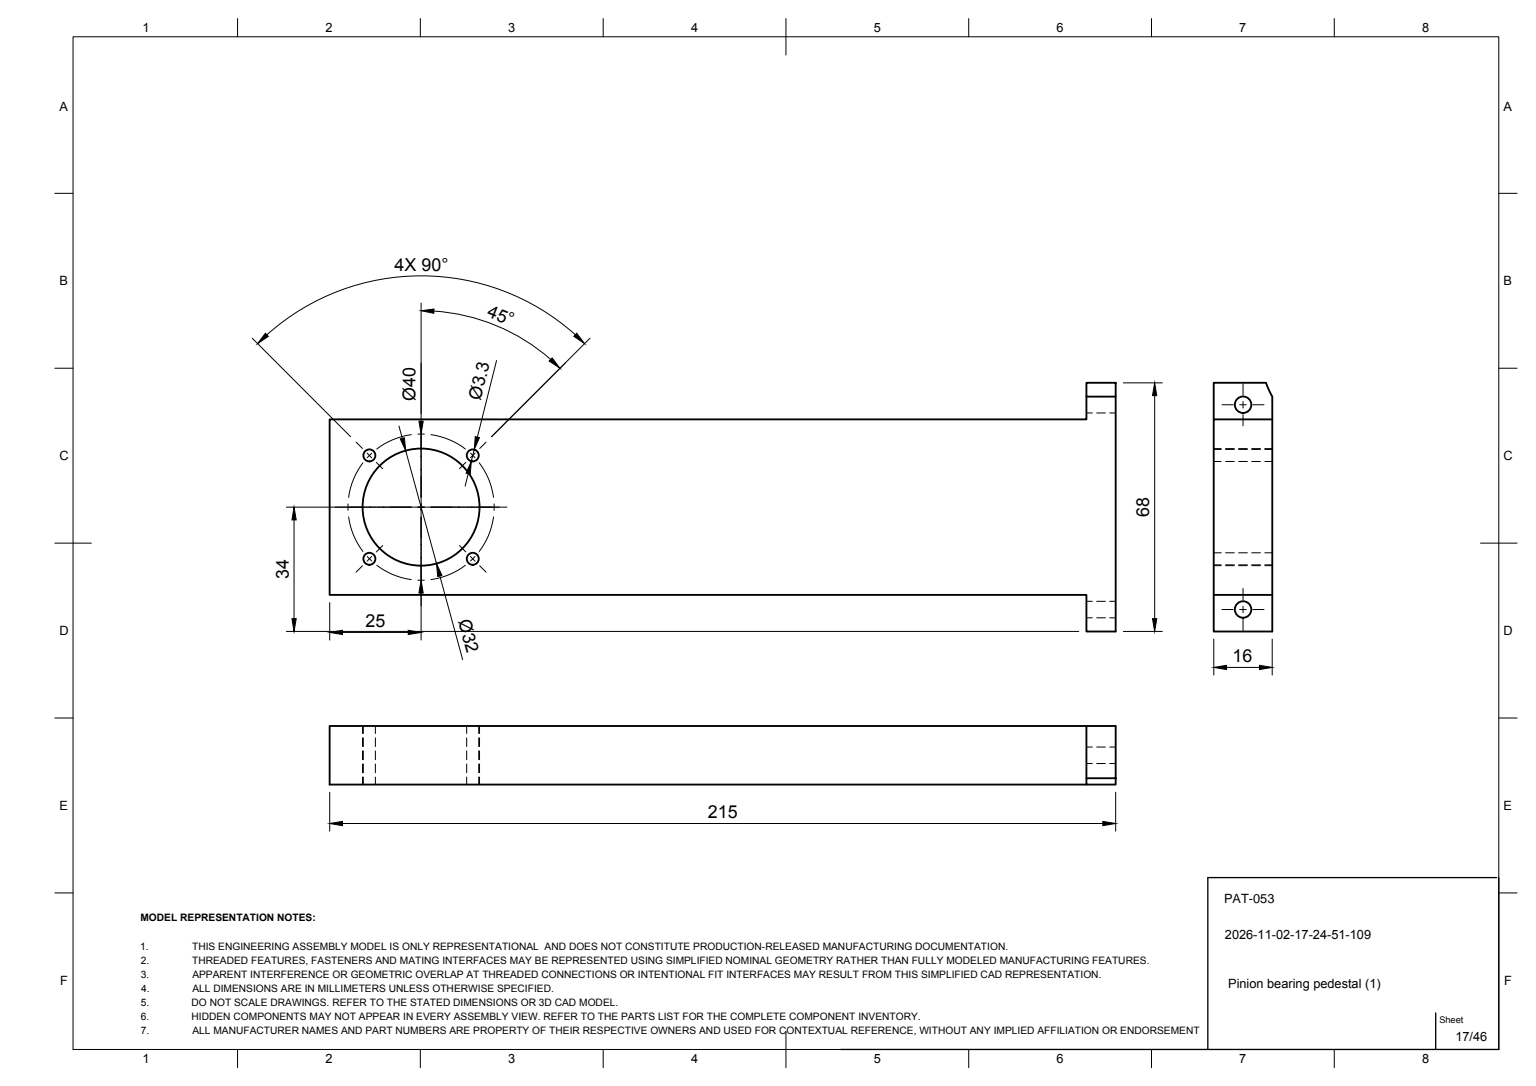
ISO-10303-21;
HEADER;
/* Generated by software containing ST-Developer
 * from STEP Tools, Inc. (www.steptools.com) 
 */

FILE_DESCRIPTION(
/* description */ ('Hand-operated arbor press'),
/* implementation_level */ '2;1');

FILE_NAME(
/* name */ 'Pinion bearing pedestal (1).step',
/* time_stamp */ '2026-10-28T03:25:25-07:00',
/* author */ (''),
/* organization */ (''),
/* preprocessor_version */ 'ST-DEVELOPER v20.2',
/* originating_system */ 'Autodesk Translation Framework v15.17.0.0',
/* authorisation */ '');

FILE_SCHEMA (('AUTOMOTIVE_DESIGN { 1 0 10303 214 3 1 1 }'));
ENDSEC;

DATA;
#10=MECHANICAL_DESIGN_GEOMETRIC_PRESENTATION_REPRESENTATION('',(#598),#32751);
#514=SHAPE_REPRESENTATION_RELATIONSHIP('SRR','None',#32943,#556);
#556=ADVANCED_BREP_SHAPE_REPRESENTATION('',(#647),#32717);
#598=STYLED_ITEM('',(#33242),#647);
#647=MANIFOLD_SOLID_BREP('Body1',#12495);
#765=FACE_BOUND('',#2225,.T.);
#766=FACE_BOUND('',#2226,.T.);
#767=FACE_BOUND('',#2228,.T.);
#768=FACE_BOUND('',#2229,.T.);
#769=FACE_BOUND('',#2230,.T.);
#770=FACE_BOUND('',#2231,.T.);
#771=FACE_BOUND('',#2232,.T.);
#772=FACE_BOUND('',#2241,.T.);
#773=FACE_BOUND('',#2243,.T.);
#774=FACE_BOUND('',#2248,.T.);
#775=FACE_BOUND('',#2249,.T.);
#776=FACE_BOUND('',#2250,.T.);
#777=FACE_BOUND('',#2251,.T.);
#778=FACE_BOUND('',#2252,.T.);
#950=PLANE('',#13307);
#951=PLANE('',#13310);
#952=PLANE('',#13330);
#953=PLANE('',#13331);
#954=PLANE('',#13332);
#955=PLANE('',#13333);
#956=PLANE('',#13334);
#957=PLANE('',#13335);
#958=PLANE('',#13336);
#959=PLANE('',#13337);
#1457=FACE_OUTER_BOUND('',#2223,.T.);
#1458=FACE_OUTER_BOUND('',#2224,.T.);
#1459=FACE_OUTER_BOUND('',#2227,.T.);
#1460=FACE_OUTER_BOUND('',#2233,.T.);
#1461=FACE_OUTER_BOUND('',#2234,.T.);
#1462=FACE_OUTER_BOUND('',#2235,.T.);
#1463=FACE_OUTER_BOUND('',#2236,.T.);
#1464=FACE_OUTER_BOUND('',#2237,.T.);
#1465=FACE_OUTER_BOUND('',#2238,.T.);
#1466=FACE_OUTER_BOUND('',#2239,.T.);
#1467=FACE_OUTER_BOUND('',#2240,.T.);
#1468=FACE_OUTER_BOUND('',#2242,.T.);
#1469=FACE_OUTER_BOUND('',#2244,.T.);
#1470=FACE_OUTER_BOUND('',#2245,.T.);
#1471=FACE_OUTER_BOUND('',#2246,.T.);
#1472=FACE_OUTER_BOUND('',#2247,.T.);
#1473=FACE_OUTER_BOUND('',#2253,.T.);
#1474=FACE_OUTER_BOUND('',#2254,.T.);
#2223=EDGE_LOOP('',(#9098,#9099,#9100,#9101));
#2224=EDGE_LOOP('',(#9102,#9103,#9104,#9105,#9106));
#2225=EDGE_LOOP('',(#9107));
#2226=EDGE_LOOP('',(#9108));
#2227=EDGE_LOOP('',(#9109,#9110,#9111,#9112,#9113,#9114,#9115,#9116));
#2228=EDGE_LOOP('',(#9117));
#2229=EDGE_LOOP('',(#9118));
#2230=EDGE_LOOP('',(#9119));
#2231=EDGE_LOOP('',(#9120));
#2232=EDGE_LOOP('',(#9121));
#2233=EDGE_LOOP('',(#9122,#9123,#9124,#9125));
#2234=EDGE_LOOP('',(#9126,#9127,#9128,#9129));
#2235=EDGE_LOOP('',(#9130,#9131,#9132,#9133));
#2236=EDGE_LOOP('',(#9134,#9135,#9136,#9137));
#2237=EDGE_LOOP('',(#9138,#9139,#9140,#9141));
#2238=EDGE_LOOP('',(#9142,#9143,#9144,#9145));
#2239=EDGE_LOOP('',(#9146,#9147,#9148,#9149));
#2240=EDGE_LOOP('',(#9150,#9151,#9152,#9153,#9154));
#2241=EDGE_LOOP('',(#9155));
#2242=EDGE_LOOP('',(#9156,#9157,#9158,#9159));
#2243=EDGE_LOOP('',(#9160));
#2244=EDGE_LOOP('',(#9161,#9162,#9163,#9164));
#2245=EDGE_LOOP('',(#9165,#9166,#9167,#9168));
#2246=EDGE_LOOP('',(#9169,#9170,#9171,#9172));
#2247=EDGE_LOOP('',(#9173,#9174,#9175,#9176,#9177,#9178,#9179,#9180));
#2248=EDGE_LOOP('',(#9181));
#2249=EDGE_LOOP('',(#9182));
#2250=EDGE_LOOP('',(#9183));
#2251=EDGE_LOOP('',(#9184));
#2252=EDGE_LOOP('',(#9185));
#2253=EDGE_LOOP('',(#9186,#9187,#9188,#9189));
#2254=EDGE_LOOP('',(#9190,#9191,#9192,#9193));
#3085=LINE('',#18467,#4256);
#3086=LINE('',#18470,#4257);
#3087=LINE('',#18473,#4258);
#3088=LINE('',#18475,#4259);
#3089=LINE('',#18477,#4260);
#3090=LINE('',#18478,#4261);
#3091=LINE('',#18485,#4262);
#3092=LINE('',#18487,#4263);
#3093=LINE('',#18489,#4264);
#3094=LINE('',#18491,#4265);
#3095=LINE('',#18493,#4266);
#3096=LINE('',#18494,#4267);
#3097=LINE('',#18507,#4268);
#3098=LINE('',#18511,#4269);
#3099=LINE('',#18515,#4270);
#3100=LINE('',#18519,#4271);
#3101=LINE('',#18523,#4272);
#3102=LINE('',#18527,#4273);
#3103=LINE('',#18531,#4274);
#3104=LINE('',#18535,#4275);
#3105=LINE('',#18537,#4276);
#3106=LINE('',#18538,#4277);
#3107=LINE('',#18541,#4278);
#3108=LINE('',#18543,#4279);
#3109=LINE('',#18544,#4280);
#3110=LINE('',#18546,#4281);
#3111=LINE('',#18548,#4282);
#3112=LINE('',#18551,#4283);
#3113=LINE('',#18552,#4284);
#3114=LINE('',#18555,#4285);
#3115=LINE('',#18556,#4286);
#3116=LINE('',#18558,#4287);
#4256=VECTOR('',#15030,1.);
#4257=VECTOR('',#15033,1.);
#4258=VECTOR('',#15036,1.);
#4259=VECTOR('',#15037,1.);
#4260=VECTOR('',#15038,1.);
#4261=VECTOR('',#15039,1.);
#4262=VECTOR('',#15046,1.);
#4263=VECTOR('',#15047,1.);
#4264=VECTOR('',#15048,1.);
#4265=VECTOR('',#15049,1.);
#4266=VECTOR('',#15050,1.);
#4267=VECTOR('',#15051,1.);
#4268=VECTOR('',#15064,0.165);
#4269=VECTOR('',#15069,0.165);
#4270=VECTOR('',#15074,0.165);
#4271=VECTOR('',#15079,0.165);
#4272=VECTOR('',#15084,0.225);
#4273=VECTOR('',#15089,0.225);
#4274=VECTOR('',#15094,1.6);
#4275=VECTOR('',#15099,1.);
#4276=VECTOR('',#15100,1.);
#4277=VECTOR('',#15101,1.);
#4278=VECTOR('',#15104,1.);
#4279=VECTOR('',#15105,1.);
#4280=VECTOR('',#15106,1.);
#4281=VECTOR('',#15109,1.);
#4282=VECTOR('',#15112,1.);
#4283=VECTOR('',#15115,1.);
#4284=VECTOR('',#15116,1.);
#4285=VECTOR('',#15119,1.);
#4286=VECTOR('',#15120,1.);
#4287=VECTOR('',#15123,1.);
#5292=CIRCLE('',#13305,2.52);
#5293=CIRCLE('',#13306,2.52);
#5294=CIRCLE('',#13308,0.225);
#5295=CIRCLE('',#13309,0.225);
#5296=CIRCLE('',#13311,0.165);
#5297=CIRCLE('',#13312,0.165);
#5298=CIRCLE('',#13313,0.165);
#5299=CIRCLE('',#13314,0.165);
#5300=CIRCLE('',#13315,1.6);
#5301=CIRCLE('',#13317,0.165);
#5302=CIRCLE('',#13319,0.165);
#5303=CIRCLE('',#13321,0.165);
#5304=CIRCLE('',#13323,0.165);
#5305=CIRCLE('',#13325,0.225);
#5306=CIRCLE('',#13327,0.225);
#5307=CIRCLE('',#13329,1.6);
#5814=VERTEX_POINT('',#18463);
#5815=VERTEX_POINT('',#18464);
#5816=VERTEX_POINT('',#18466);
#5817=VERTEX_POINT('',#18468);
#5818=VERTEX_POINT('',#18472);
#5819=VERTEX_POINT('',#18474);
#5820=VERTEX_POINT('',#18476);
#5821=VERTEX_POINT('',#18479);
#5822=VERTEX_POINT('',#18481);
#5823=VERTEX_POINT('',#18484);
#5824=VERTEX_POINT('',#18486);
#5825=VERTEX_POINT('',#18488);
#5826=VERTEX_POINT('',#18490);
#5827=VERTEX_POINT('',#18492);
#5828=VERTEX_POINT('',#18495);
#5829=VERTEX_POINT('',#18497);
#5830=VERTEX_POINT('',#18499);
#5831=VERTEX_POINT('',#18501);
#5832=VERTEX_POINT('',#18503);
#5833=VERTEX_POINT('',#18506);
#5834=VERTEX_POINT('',#18510);
#5835=VERTEX_POINT('',#18514);
#5836=VERTEX_POINT('',#18518);
#5837=VERTEX_POINT('',#18522);
#5838=VERTEX_POINT('',#18526);
#5839=VERTEX_POINT('',#18530);
#5840=VERTEX_POINT('',#18534);
#5841=VERTEX_POINT('',#18536);
#5842=VERTEX_POINT('',#18540);
#5843=VERTEX_POINT('',#18542);
#5844=VERTEX_POINT('',#18550);
#5845=VERTEX_POINT('',#18554);
#7052=EDGE_CURVE('',#5814,#5815,#5292,.T.);
#7053=EDGE_CURVE('',#5816,#5814,#3085,.T.);
#7054=EDGE_CURVE('',#5817,#5816,#5293,.T.);
#7055=EDGE_CURVE('',#5815,#5817,#3086,.T.);
#7056=EDGE_CURVE('',#5818,#5816,#3087,.T.);
#7057=EDGE_CURVE('',#5818,#5819,#3088,.T.);
#7058=EDGE_CURVE('',#5820,#5819,#3089,.T.);
#7059=EDGE_CURVE('',#5817,#5820,#3090,.T.);
#7060=EDGE_CURVE('',#5821,#5821,#5294,.T.);
#7061=EDGE_CURVE('',#5822,#5822,#5295,.T.);
#7062=EDGE_CURVE('',#5814,#5823,#3091,.T.);
#7063=EDGE_CURVE('',#5823,#5824,#3092,.T.);
#7064=EDGE_CURVE('',#5825,#5824,#3093,.T.);
#7065=EDGE_CURVE('',#5826,#5825,#3094,.T.);
#7066=EDGE_CURVE('',#5826,#5827,#3095,.T.);
#7067=EDGE_CURVE('',#5827,#5818,#3096,.T.);
#7068=EDGE_CURVE('',#5828,#5828,#5296,.T.);
#7069=EDGE_CURVE('',#5829,#5829,#5297,.T.);
#7070=EDGE_CURVE('',#5830,#5830,#5298,.T.);
#7071=EDGE_CURVE('',#5831,#5831,#5299,.T.);
#7072=EDGE_CURVE('',#5832,#5832,#5300,.T.);
#7073=EDGE_CURVE('',#5828,#5833,#3097,.T.);
#7074=EDGE_CURVE('',#5833,#5833,#5301,.T.);
#7075=EDGE_CURVE('',#5829,#5834,#3098,.T.);
#7076=EDGE_CURVE('',#5834,#5834,#5302,.T.);
#7077=EDGE_CURVE('',#5830,#5835,#3099,.T.);
#7078=EDGE_CURVE('',#5835,#5835,#5303,.T.);
#7079=EDGE_CURVE('',#5831,#5836,#3100,.T.);
#7080=EDGE_CURVE('',#5836,#5836,#5304,.T.);
#7081=EDGE_CURVE('',#5822,#5837,#3101,.T.);
#7082=EDGE_CURVE('',#5837,#5837,#5305,.T.);
#7083=EDGE_CURVE('',#5821,#5838,#3102,.T.);
#7084=EDGE_CURVE('',#5838,#5838,#5306,.T.);
#7085=EDGE_CURVE('',#5832,#5839,#3103,.T.);
#7086=EDGE_CURVE('',#5839,#5839,#5307,.T.);
#7087=EDGE_CURVE('',#5815,#5840,#3104,.T.);
#7088=EDGE_CURVE('',#5841,#5840,#3105,.T.);
#7089=EDGE_CURVE('',#5823,#5841,#3106,.T.);
#7090=EDGE_CURVE('',#5842,#5826,#3107,.T.);
#7091=EDGE_CURVE('',#5843,#5842,#3108,.T.);
#7092=EDGE_CURVE('',#5827,#5843,#3109,.T.);
#7093=EDGE_CURVE('',#5819,#5843,#3110,.T.);
#7094=EDGE_CURVE('',#5840,#5820,#3111,.T.);
#7095=EDGE_CURVE('',#5841,#5844,#3112,.T.);
#7096=EDGE_CURVE('',#5824,#5844,#3113,.T.);
#7097=EDGE_CURVE('',#5842,#5845,#3114,.T.);
#7098=EDGE_CURVE('',#5844,#5845,#3115,.T.);
#7099=EDGE_CURVE('',#5845,#5825,#3116,.T.);
#9098=ORIENTED_EDGE('',*,*,#7052,.F.);
#9099=ORIENTED_EDGE('',*,*,#7053,.F.);
#9100=ORIENTED_EDGE('',*,*,#7054,.F.);
#9101=ORIENTED_EDGE('',*,*,#7055,.F.);
#9102=ORIENTED_EDGE('',*,*,#7054,.T.);
#9103=ORIENTED_EDGE('',*,*,#7056,.F.);
#9104=ORIENTED_EDGE('',*,*,#7057,.T.);
#9105=ORIENTED_EDGE('',*,*,#7058,.F.);
#9106=ORIENTED_EDGE('',*,*,#7059,.F.);
#9107=ORIENTED_EDGE('',*,*,#7060,.T.);
#9108=ORIENTED_EDGE('',*,*,#7061,.T.);
#9109=ORIENTED_EDGE('',*,*,#7053,.T.);
#9110=ORIENTED_EDGE('',*,*,#7062,.T.);
#9111=ORIENTED_EDGE('',*,*,#7063,.T.);
#9112=ORIENTED_EDGE('',*,*,#7064,.F.);
#9113=ORIENTED_EDGE('',*,*,#7065,.F.);
#9114=ORIENTED_EDGE('',*,*,#7066,.T.);
#9115=ORIENTED_EDGE('',*,*,#7067,.T.);
#9116=ORIENTED_EDGE('',*,*,#7056,.T.);
#9117=ORIENTED_EDGE('',*,*,#7068,.T.);
#9118=ORIENTED_EDGE('',*,*,#7069,.T.);
#9119=ORIENTED_EDGE('',*,*,#7070,.T.);
#9120=ORIENTED_EDGE('',*,*,#7071,.T.);
#9121=ORIENTED_EDGE('',*,*,#7072,.T.);
#9122=ORIENTED_EDGE('',*,*,#7068,.F.);
#9123=ORIENTED_EDGE('',*,*,#7073,.T.);
#9124=ORIENTED_EDGE('',*,*,#7074,.F.);
#9125=ORIENTED_EDGE('',*,*,#7073,.F.);
#9126=ORIENTED_EDGE('',*,*,#7069,.F.);
#9127=ORIENTED_EDGE('',*,*,#7075,.T.);
#9128=ORIENTED_EDGE('',*,*,#7076,.F.);
#9129=ORIENTED_EDGE('',*,*,#7075,.F.);
#9130=ORIENTED_EDGE('',*,*,#7070,.F.);
#9131=ORIENTED_EDGE('',*,*,#7077,.T.);
#9132=ORIENTED_EDGE('',*,*,#7078,.F.);
#9133=ORIENTED_EDGE('',*,*,#7077,.F.);
#9134=ORIENTED_EDGE('',*,*,#7071,.F.);
#9135=ORIENTED_EDGE('',*,*,#7079,.T.);
#9136=ORIENTED_EDGE('',*,*,#7080,.F.);
#9137=ORIENTED_EDGE('',*,*,#7079,.F.);
#9138=ORIENTED_EDGE('',*,*,#7061,.F.);
#9139=ORIENTED_EDGE('',*,*,#7081,.T.);
#9140=ORIENTED_EDGE('',*,*,#7082,.F.);
#9141=ORIENTED_EDGE('',*,*,#7081,.F.);
#9142=ORIENTED_EDGE('',*,*,#7060,.F.);
#9143=ORIENTED_EDGE('',*,*,#7083,.T.);
#9144=ORIENTED_EDGE('',*,*,#7084,.F.);
#9145=ORIENTED_EDGE('',*,*,#7083,.F.);
#9146=ORIENTED_EDGE('',*,*,#7072,.F.);
#9147=ORIENTED_EDGE('',*,*,#7085,.T.);
#9148=ORIENTED_EDGE('',*,*,#7086,.F.);
#9149=ORIENTED_EDGE('',*,*,#7085,.F.);
#9150=ORIENTED_EDGE('',*,*,#7052,.T.);
#9151=ORIENTED_EDGE('',*,*,#7087,.T.);
#9152=ORIENTED_EDGE('',*,*,#7088,.F.);
#9153=ORIENTED_EDGE('',*,*,#7089,.F.);
#9154=ORIENTED_EDGE('',*,*,#7062,.F.);
#9155=ORIENTED_EDGE('',*,*,#7084,.T.);
#9156=ORIENTED_EDGE('',*,*,#7090,.F.);
#9157=ORIENTED_EDGE('',*,*,#7091,.F.);
#9158=ORIENTED_EDGE('',*,*,#7092,.F.);
#9159=ORIENTED_EDGE('',*,*,#7066,.F.);
#9160=ORIENTED_EDGE('',*,*,#7082,.T.);
#9161=ORIENTED_EDGE('',*,*,#7067,.F.);
#9162=ORIENTED_EDGE('',*,*,#7092,.T.);
#9163=ORIENTED_EDGE('',*,*,#7093,.F.);
#9164=ORIENTED_EDGE('',*,*,#7057,.F.);
#9165=ORIENTED_EDGE('',*,*,#7055,.T.);
#9166=ORIENTED_EDGE('',*,*,#7059,.T.);
#9167=ORIENTED_EDGE('',*,*,#7094,.F.);
#9168=ORIENTED_EDGE('',*,*,#7087,.F.);
#9169=ORIENTED_EDGE('',*,*,#7089,.T.);
#9170=ORIENTED_EDGE('',*,*,#7095,.T.);
#9171=ORIENTED_EDGE('',*,*,#7096,.F.);
#9172=ORIENTED_EDGE('',*,*,#7063,.F.);
#9173=ORIENTED_EDGE('',*,*,#7097,.T.);
#9174=ORIENTED_EDGE('',*,*,#7098,.F.);
#9175=ORIENTED_EDGE('',*,*,#7095,.F.);
#9176=ORIENTED_EDGE('',*,*,#7088,.T.);
#9177=ORIENTED_EDGE('',*,*,#7094,.T.);
#9178=ORIENTED_EDGE('',*,*,#7058,.T.);
#9179=ORIENTED_EDGE('',*,*,#7093,.T.);
#9180=ORIENTED_EDGE('',*,*,#7091,.T.);
#9181=ORIENTED_EDGE('',*,*,#7086,.T.);
#9182=ORIENTED_EDGE('',*,*,#7080,.T.);
#9183=ORIENTED_EDGE('',*,*,#7078,.T.);
#9184=ORIENTED_EDGE('',*,*,#7076,.T.);
#9185=ORIENTED_EDGE('',*,*,#7074,.T.);
#9186=ORIENTED_EDGE('',*,*,#7090,.T.);
#9187=ORIENTED_EDGE('',*,*,#7065,.T.);
#9188=ORIENTED_EDGE('',*,*,#7099,.F.);
#9189=ORIENTED_EDGE('',*,*,#7097,.F.);
#9190=ORIENTED_EDGE('',*,*,#7099,.T.);
#9191=ORIENTED_EDGE('',*,*,#7064,.T.);
#9192=ORIENTED_EDGE('',*,*,#7096,.T.);
#9193=ORIENTED_EDGE('',*,*,#7098,.T.);
#11705=CYLINDRICAL_SURFACE('',#13304,2.52);
#11706=CYLINDRICAL_SURFACE('',#13316,0.165);
#11707=CYLINDRICAL_SURFACE('',#13318,0.165);
#11708=CYLINDRICAL_SURFACE('',#13320,0.165);
#11709=CYLINDRICAL_SURFACE('',#13322,0.165);
#11710=CYLINDRICAL_SURFACE('',#13324,0.225);
#11711=CYLINDRICAL_SURFACE('',#13326,0.225);
#11712=CYLINDRICAL_SURFACE('',#13328,1.6);
#11966=ADVANCED_FACE('',(#1457),#11705,.F.);
#11967=ADVANCED_FACE('',(#1458,#765,#766),#950,.F.);
#11968=ADVANCED_FACE('',(#1459,#767,#768,#769,#770,#771),#951,.T.);
#11969=ADVANCED_FACE('',(#1460),#11706,.F.);
#11970=ADVANCED_FACE('',(#1461),#11707,.F.);
#11971=ADVANCED_FACE('',(#1462),#11708,.F.);
#11972=ADVANCED_FACE('',(#1463),#11709,.F.);
#11973=ADVANCED_FACE('',(#1464),#11710,.F.);
#11974=ADVANCED_FACE('',(#1465),#11711,.F.);
#11975=ADVANCED_FACE('',(#1466),#11712,.F.);
#11976=ADVANCED_FACE('',(#1467,#772),#952,.T.);
#11977=ADVANCED_FACE('',(#1468,#773),#953,.T.);
#11978=ADVANCED_FACE('',(#1469),#954,.T.);
#11979=ADVANCED_FACE('',(#1470),#955,.T.);
#11980=ADVANCED_FACE('',(#1471),#956,.T.);
#11981=ADVANCED_FACE('',(#1472,#774,#775,#776,#777,#778),#957,.T.);
#11982=ADVANCED_FACE('',(#1473),#958,.T.);
#11983=ADVANCED_FACE('',(#1474),#959,.T.);
#12495=CLOSED_SHELL('',(#11966,#11967,#11968,#11969,#11970,#11971,#11972,
#11973,#11974,#11975,#11976,#11977,#11978,#11979,#11980,#11981,#11982,#11983));
#13303=AXIS2_PLACEMENT_3D('',#18461,#15024,#15025);
#13304=AXIS2_PLACEMENT_3D('',#18462,#15026,#15027);
#13305=AXIS2_PLACEMENT_3D('',#18465,#15028,#15029);
#13306=AXIS2_PLACEMENT_3D('',#18469,#15031,#15032);
#13307=AXIS2_PLACEMENT_3D('',#18471,#15034,#15035);
#13308=AXIS2_PLACEMENT_3D('',#18480,#15040,#15041);
#13309=AXIS2_PLACEMENT_3D('',#18482,#15042,#15043);
#13310=AXIS2_PLACEMENT_3D('',#18483,#15044,#15045);
#13311=AXIS2_PLACEMENT_3D('',#18496,#15052,#15053);
#13312=AXIS2_PLACEMENT_3D('',#18498,#15054,#15055);
#13313=AXIS2_PLACEMENT_3D('',#18500,#15056,#15057);
#13314=AXIS2_PLACEMENT_3D('',#18502,#15058,#15059);
#13315=AXIS2_PLACEMENT_3D('',#18504,#15060,#15061);
#13316=AXIS2_PLACEMENT_3D('',#18505,#15062,#15063);
#13317=AXIS2_PLACEMENT_3D('',#18508,#15065,#15066);
#13318=AXIS2_PLACEMENT_3D('',#18509,#15067,#15068);
#13319=AXIS2_PLACEMENT_3D('',#18512,#15070,#15071);
#13320=AXIS2_PLACEMENT_3D('',#18513,#15072,#15073);
#13321=AXIS2_PLACEMENT_3D('',#18516,#15075,#15076);
#13322=AXIS2_PLACEMENT_3D('',#18517,#15077,#15078);
#13323=AXIS2_PLACEMENT_3D('',#18520,#15080,#15081);
#13324=AXIS2_PLACEMENT_3D('',#18521,#15082,#15083);
#13325=AXIS2_PLACEMENT_3D('',#18524,#15085,#15086);
#13326=AXIS2_PLACEMENT_3D('',#18525,#15087,#15088);
#13327=AXIS2_PLACEMENT_3D('',#18528,#15090,#15091);
#13328=AXIS2_PLACEMENT_3D('',#18529,#15092,#15093);
#13329=AXIS2_PLACEMENT_3D('',#18532,#15095,#15096);
#13330=AXIS2_PLACEMENT_3D('',#18533,#15097,#15098);
#13331=AXIS2_PLACEMENT_3D('',#18539,#15102,#15103);
#13332=AXIS2_PLACEMENT_3D('',#18545,#15107,#15108);
#13333=AXIS2_PLACEMENT_3D('',#18547,#15110,#15111);
#13334=AXIS2_PLACEMENT_3D('',#18549,#15113,#15114);
#13335=AXIS2_PLACEMENT_3D('',#18553,#15117,#15118);
#13336=AXIS2_PLACEMENT_3D('',#18557,#15121,#15122);
#13337=AXIS2_PLACEMENT_3D('',#18559,#15124,#15125);
#15024=DIRECTION('axis',(0.,0.,1.));
#15025=DIRECTION('refdir',(1.,0.,0.));
#15026=DIRECTION('center_axis',(0.,0.,1.));
#15027=DIRECTION('ref_axis',(1.,0.,0.));
#15028=DIRECTION('center_axis',(0.,0.,-1.));
#15029=DIRECTION('ref_axis',(1.,0.,0.));
#15030=DIRECTION('',(0.,0.,1.));
#15031=DIRECTION('center_axis',(0.,0.,1.));
#15032=DIRECTION('ref_axis',(1.,0.,0.));
#15033=DIRECTION('',(0.,0.,-1.));
#15034=DIRECTION('center_axis',(0.,0.,1.));
#15035=DIRECTION('ref_axis',(1.,0.,0.));
#15036=DIRECTION('',(1.,0.,0.));
#15037=DIRECTION('',(0.,1.,0.));
#15038=DIRECTION('',(-1.,0.,0.));
#15039=DIRECTION('',(0.,1.,0.));
#15040=DIRECTION('center_axis',(0.,0.,1.));
#15041=DIRECTION('ref_axis',(1.,0.,0.));
#15042=DIRECTION('center_axis',(0.,0.,1.));
#15043=DIRECTION('ref_axis',(1.,0.,0.));
#15044=DIRECTION('center_axis',(0.,-1.,0.));
#15045=DIRECTION('ref_axis',(1.,0.,0.));
#15046=DIRECTION('',(-1.,0.,0.));
#15047=DIRECTION('',(0.,0.,1.));
#15048=DIRECTION('',(1.,0.,0.));
#15049=DIRECTION('',(0.,0.,1.));
#15050=DIRECTION('',(-1.,0.,0.));
#15051=DIRECTION('',(0.,0.,-1.));
#15052=DIRECTION('center_axis',(0.,1.,0.));
#15053=DIRECTION('ref_axis',(1.,0.,0.));
#15054=DIRECTION('center_axis',(0.,1.,0.));
#15055=DIRECTION('ref_axis',(1.,0.,0.));
#15056=DIRECTION('center_axis',(0.,1.,0.));
#15057=DIRECTION('ref_axis',(1.,0.,0.));
#15058=DIRECTION('center_axis',(0.,1.,0.));
#15059=DIRECTION('ref_axis',(1.,0.,0.));
#15060=DIRECTION('center_axis',(0.,1.,0.));
#15061=DIRECTION('ref_axis',(1.,0.,0.));
#15062=DIRECTION('center_axis',(0.,1.,0.));
#15063=DIRECTION('ref_axis',(1.,0.,0.));
#15064=DIRECTION('',(0.,1.,0.));
#15065=DIRECTION('center_axis',(0.,-1.,0.));
#15066=DIRECTION('ref_axis',(1.,0.,0.));
#15067=DIRECTION('center_axis',(0.,1.,0.));
#15068=DIRECTION('ref_axis',(1.,0.,0.));
#15069=DIRECTION('',(0.,1.,0.));
#15070=DIRECTION('center_axis',(0.,-1.,0.));
#15071=DIRECTION('ref_axis',(1.,0.,0.));
#15072=DIRECTION('center_axis',(0.,1.,0.));
#15073=DIRECTION('ref_axis',(1.,0.,0.));
#15074=DIRECTION('',(0.,1.,0.));
#15075=DIRECTION('center_axis',(0.,-1.,0.));
#15076=DIRECTION('ref_axis',(1.,0.,0.));
#15077=DIRECTION('center_axis',(0.,1.,0.));
#15078=DIRECTION('ref_axis',(1.,0.,0.));
#15079=DIRECTION('',(0.,1.,0.));
#15080=DIRECTION('center_axis',(0.,-1.,0.));
#15081=DIRECTION('ref_axis',(1.,0.,0.));
#15082=DIRECTION('center_axis',(0.,0.,1.));
#15083=DIRECTION('ref_axis',(1.,0.,0.));
#15084=DIRECTION('',(0.,0.,1.));
#15085=DIRECTION('center_axis',(0.,0.,-1.));
#15086=DIRECTION('ref_axis',(1.,0.,0.));
#15087=DIRECTION('center_axis',(0.,0.,1.));
#15088=DIRECTION('ref_axis',(1.,0.,0.));
#15089=DIRECTION('',(0.,0.,1.));
#15090=DIRECTION('center_axis',(0.,0.,-1.));
#15091=DIRECTION('ref_axis',(1.,0.,0.));
#15092=DIRECTION('center_axis',(0.,1.,0.));
#15093=DIRECTION('ref_axis',(1.,0.,0.));
#15094=DIRECTION('',(0.,1.,0.));
#15095=DIRECTION('center_axis',(0.,-1.,0.));
#15096=DIRECTION('ref_axis',(1.,0.,0.));
#15097=DIRECTION('center_axis',(0.,0.,1.));
#15098=DIRECTION('ref_axis',(1.,0.,0.));
#15099=DIRECTION('',(0.,1.,0.));
#15100=DIRECTION('',(1.,0.,0.));
#15101=DIRECTION('',(0.,1.,0.));
#15102=DIRECTION('center_axis',(0.,0.,1.));
#15103=DIRECTION('ref_axis',(1.,0.,0.));
#15104=DIRECTION('',(0.,-1.,0.));
#15105=DIRECTION('',(1.,0.,0.));
#15106=DIRECTION('',(0.,1.,0.));
#15107=DIRECTION('center_axis',(-1.,0.,0.));
#15108=DIRECTION('ref_axis',(0.,0.,1.));
#15109=DIRECTION('',(0.,0.,1.));
#15110=DIRECTION('center_axis',(1.,0.,0.));
#15111=DIRECTION('ref_axis',(0.,0.,-1.));
#15112=DIRECTION('',(0.,0.,-1.));
#15113=DIRECTION('center_axis',(1.,0.,0.));
#15114=DIRECTION('ref_axis',(0.,1.,0.));
#15115=DIRECTION('',(0.,0.,1.));
#15116=DIRECTION('',(0.,1.,0.));
#15117=DIRECTION('center_axis',(0.,1.,0.));
#15118=DIRECTION('ref_axis',(-1.,0.,0.));
#15119=DIRECTION('',(0.,0.,1.));
#15120=DIRECTION('',(-1.,0.,0.));
#15121=DIRECTION('center_axis',(-1.,0.,0.));
#15122=DIRECTION('ref_axis',(0.,-1.,0.));
#15123=DIRECTION('',(0.,-1.,0.));
#15124=DIRECTION('center_axis',(0.,0.,1.));
#15125=DIRECTION('ref_axis',(1.,0.,0.));
#18461=CARTESIAN_POINT('',(0.,0.,0.));
#18462=CARTESIAN_POINT('Origin',(1.,0.,0.9));
#18463=CARTESIAN_POINT('',(-0.228983319658977,2.2,1.8));
#18464=CARTESIAN_POINT('',(0.15,2.37231954002828,1.8));
#18465=CARTESIAN_POINT('Origin',(1.,0.,1.8));
#18466=CARTESIAN_POINT('',(-0.228983319658977,2.2,1.));
#18467=CARTESIAN_POINT('',(-0.228983319658977,2.2,0.9));
#18468=CARTESIAN_POINT('',(0.15,2.37231954002828,1.));
#18469=CARTESIAN_POINT('Origin',(1.,0.,1.));
#18470=CARTESIAN_POINT('',(0.15,2.37231954002828,0.9));
#18471=CARTESIAN_POINT('Origin',(-3.25,3.,1.));
#18472=CARTESIAN_POINT('',(-6.65,2.2,1.));
#18473=CARTESIAN_POINT('',(-6.65,2.2,1.));
#18474=CARTESIAN_POINT('',(-6.65,3.8,1.));
#18475=CARTESIAN_POINT('',(-6.65,2.2,1.));
#18476=CARTESIAN_POINT('',(0.15,3.8,1.));
#18477=CARTESIAN_POINT('',(-6.65,3.8,1.));
#18478=CARTESIAN_POINT('',(0.15,2.2,1.));
#18479=CARTESIAN_POINT('',(-0.675,3.,1.));
#18480=CARTESIAN_POINT('Origin',(-0.45,3.,1.));
#18481=CARTESIAN_POINT('',(-6.275,3.,1.));
#18482=CARTESIAN_POINT('Origin',(-6.05,3.,1.));
#18483=CARTESIAN_POINT('Origin',(-5.65,2.2,1.));
#18484=CARTESIAN_POINT('',(-0.85,2.2,1.8));
#18485=CARTESIAN_POINT('',(0.15,2.2,1.8));
#18486=CARTESIAN_POINT('',(-0.85,2.2,22.5));
#18487=CARTESIAN_POINT('',(-0.85,2.2,1.));
#18488=CARTESIAN_POINT('',(-5.65,2.2,22.5));
#18489=CARTESIAN_POINT('',(-5.65,2.2,22.5));
#18490=CARTESIAN_POINT('',(-5.65,2.2,1.8));
#18491=CARTESIAN_POINT('',(-5.65,2.2,1.));
#18492=CARTESIAN_POINT('',(-6.65,2.2,1.8));
#18493=CARTESIAN_POINT('',(0.15,2.2,1.8));
#18494=CARTESIAN_POINT('',(-6.65,2.2,1.8));
#18495=CARTESIAN_POINT('',(-4.82921356237309,2.2,18.5857864376269));
#18496=CARTESIAN_POINT('Origin',(-4.66421356237309,2.2,18.5857864376269));
#18497=CARTESIAN_POINT('',(-4.82921356237309,2.2,21.4142135623731));
#18498=CARTESIAN_POINT('Origin',(-4.66421356237309,2.2,21.4142135623731));
#18499=CARTESIAN_POINT('',(-2.00078643762691,2.2,21.4142135623731));
#18500=CARTESIAN_POINT('Origin',(-1.8357864376269,2.2,21.4142135623731));
#18501=CARTESIAN_POINT('',(-2.00078643762691,2.2,18.5857864376269));
#18502=CARTESIAN_POINT('Origin',(-1.83578643762691,2.2,18.5857864376269));
#18503=CARTESIAN_POINT('',(-4.85,2.2,20.));
#18504=CARTESIAN_POINT('Origin',(-3.25,2.2,20.));
#18505=CARTESIAN_POINT('Origin',(-4.66421356237309,2.1,18.5857864376269));
#18506=CARTESIAN_POINT('',(-4.82921356237309,3.8,18.5857864376269));
#18507=CARTESIAN_POINT('',(-4.82921356237309,2.1,18.5857864376269));
#18508=CARTESIAN_POINT('Origin',(-4.66421356237309,3.8,18.5857864376269));
#18509=CARTESIAN_POINT('Origin',(-4.66421356237309,2.1,21.4142135623731));
#18510=CARTESIAN_POINT('',(-4.82921356237309,3.8,21.4142135623731));
#18511=CARTESIAN_POINT('',(-4.82921356237309,2.1,21.4142135623731));
#18512=CARTESIAN_POINT('Origin',(-4.66421356237309,3.8,21.4142135623731));
#18513=CARTESIAN_POINT('Origin',(-1.8357864376269,2.1,21.4142135623731));
#18514=CARTESIAN_POINT('',(-2.00078643762691,3.8,21.4142135623731));
#18515=CARTESIAN_POINT('',(-2.00078643762691,2.1,21.4142135623731));
#18516=CARTESIAN_POINT('Origin',(-1.8357864376269,3.8,21.4142135623731));
#18517=CARTESIAN_POINT('Origin',(-1.83578643762691,2.1,18.5857864376269));
#18518=CARTESIAN_POINT('',(-2.00078643762691,3.8,18.5857864376269));
#18519=CARTESIAN_POINT('',(-2.00078643762691,2.1,18.5857864376269));
#18520=CARTESIAN_POINT('Origin',(-1.83578643762691,3.8,18.5857864376269));
#18521=CARTESIAN_POINT('Origin',(-6.05,3.,0.9));
#18522=CARTESIAN_POINT('',(-6.275,3.,1.8));
#18523=CARTESIAN_POINT('',(-6.275,3.,0.9));
#18524=CARTESIAN_POINT('Origin',(-6.05,3.,1.8));
#18525=CARTESIAN_POINT('Origin',(-0.45,3.,0.9));
#18526=CARTESIAN_POINT('',(-0.675,3.,1.8));
#18527=CARTESIAN_POINT('',(-0.675,3.,0.9));
#18528=CARTESIAN_POINT('Origin',(-0.45,3.,1.8));
#18529=CARTESIAN_POINT('Origin',(-3.25,2.1,20.));
#18530=CARTESIAN_POINT('',(-4.85,3.8,20.));
#18531=CARTESIAN_POINT('',(-4.85,2.1,20.));
#18532=CARTESIAN_POINT('Origin',(-3.25,3.8,20.));
#18533=CARTESIAN_POINT('Origin',(-6.65,2.2,1.8));
#18534=CARTESIAN_POINT('',(0.15,3.8,1.8));
#18535=CARTESIAN_POINT('',(0.15,2.2,1.8));
#18536=CARTESIAN_POINT('',(-0.85,3.8,1.8));
#18537=CARTESIAN_POINT('',(0.15,3.8,1.8));
#18538=CARTESIAN_POINT('',(-0.85,2.2,1.8));
#18539=CARTESIAN_POINT('Origin',(-6.65,2.2,1.8));
#18540=CARTESIAN_POINT('',(-5.65,3.8,1.8));
#18541=CARTESIAN_POINT('',(-5.65,3.,1.8));
#18542=CARTESIAN_POINT('',(-6.65,3.8,1.8));
#18543=CARTESIAN_POINT('',(0.15,3.8,1.8));
#18544=CARTESIAN_POINT('',(-6.65,2.2,1.8));
#18545=CARTESIAN_POINT('Origin',(-6.65,2.2,1.));
#18546=CARTESIAN_POINT('',(-6.65,3.8,1.8));
#18547=CARTESIAN_POINT('Origin',(0.15,2.2,1.8));
#18548=CARTESIAN_POINT('',(0.15,3.8,1.));
#18549=CARTESIAN_POINT('Origin',(-0.85,2.2,1.));
#18550=CARTESIAN_POINT('',(-0.85,3.8,22.5));
#18551=CARTESIAN_POINT('',(-0.85,3.8,1.));
#18552=CARTESIAN_POINT('',(-0.85,2.2,22.5));
#18553=CARTESIAN_POINT('Origin',(-0.85,3.8,1.));
#18554=CARTESIAN_POINT('',(-5.65,3.8,22.5));
#18555=CARTESIAN_POINT('',(-5.65,3.8,1.));
#18556=CARTESIAN_POINT('',(-0.85,3.8,22.5));
#18557=CARTESIAN_POINT('Origin',(-5.65,3.8,1.));
#18558=CARTESIAN_POINT('',(-5.65,3.8,22.5));
#18559=CARTESIAN_POINT('Origin',(-3.25,3.,22.5));
#32668=UNCERTAINTY_MEASURE_WITH_UNIT(LENGTH_MEASURE(0.001),#32752,
'DISTANCE_ACCURACY_VALUE',
'Maximum model space distance between geometric entities at asserted c
onnectivities');
#32702=UNCERTAINTY_MEASURE_WITH_UNIT(LENGTH_MEASURE(0.001),#32752,
'DISTANCE_ACCURACY_VALUE',
'Maximum model space distance between geometric entities at asserted c
onnectivities');
#32717=(
GEOMETRIC_REPRESENTATION_CONTEXT(3)
GLOBAL_UNCERTAINTY_ASSIGNED_CONTEXT((#32668))
GLOBAL_UNIT_ASSIGNED_CONTEXT((#32752,#32754,#32755))
REPRESENTATION_CONTEXT('','3D')
);
#32751=(
GEOMETRIC_REPRESENTATION_CONTEXT(3)
GLOBAL_UNCERTAINTY_ASSIGNED_CONTEXT((#32702))
GLOBAL_UNIT_ASSIGNED_CONTEXT((#32752,#32754,#32755))
REPRESENTATION_CONTEXT('','3D')
);
#32752=(
LENGTH_UNIT()
NAMED_UNIT(*)
SI_UNIT(.CENTI.,.METRE.)
);
#32754=(
NAMED_UNIT(*)
PLANE_ANGLE_UNIT()
SI_UNIT($,.RADIAN.)
);
#32755=(
NAMED_UNIT(*)
SI_UNIT($,.STERADIAN.)
SOLID_ANGLE_UNIT()
);
#32770=SHAPE_DEFINITION_REPRESENTATION(#32818,#32943);
#32818=PRODUCT_DEFINITION_SHAPE('',$,#32992);
#32943=SHAPE_REPRESENTATION('',(#13303),#32717);
#32977=PRODUCT_DEFINITION_CONTEXT('part definition',#33123,'design');
#32992=PRODUCT_DEFINITION('Pinion bearing pedestal (1)',
'Pinion bearing pedestal (1)',#33040,#32977);
#33040=PRODUCT_DEFINITION_FORMATION('',$,#33139);
#33123=APPLICATION_CONTEXT(
'Core Data for Automotive Mechanical Design Process');
#33124=PRODUCT_CONTEXT('part definition',#33123,'mechanical');
#33139=PRODUCT('Pinion bearing pedestal (1)',
'Pinion bearing pedestal (1)','Pinion bearing pedestal (1)',(#33124));
#33236=COLOUR_RGB('Grey',0.48,0.52,0.57);
#33237=FILL_AREA_STYLE_COLOUR('',#33236);
#33238=FILL_AREA_STYLE('',(#33237));
#33239=SURFACE_STYLE_FILL_AREA(#33238);
#33240=SURFACE_SIDE_STYLE('',(#33239));
#33241=SURFACE_STYLE_USAGE(.BOTH.,#33240);
#33242=PRESENTATION_STYLE_ASSIGNMENT((#33241));
ENDSEC;
END-ISO-10303-21;
